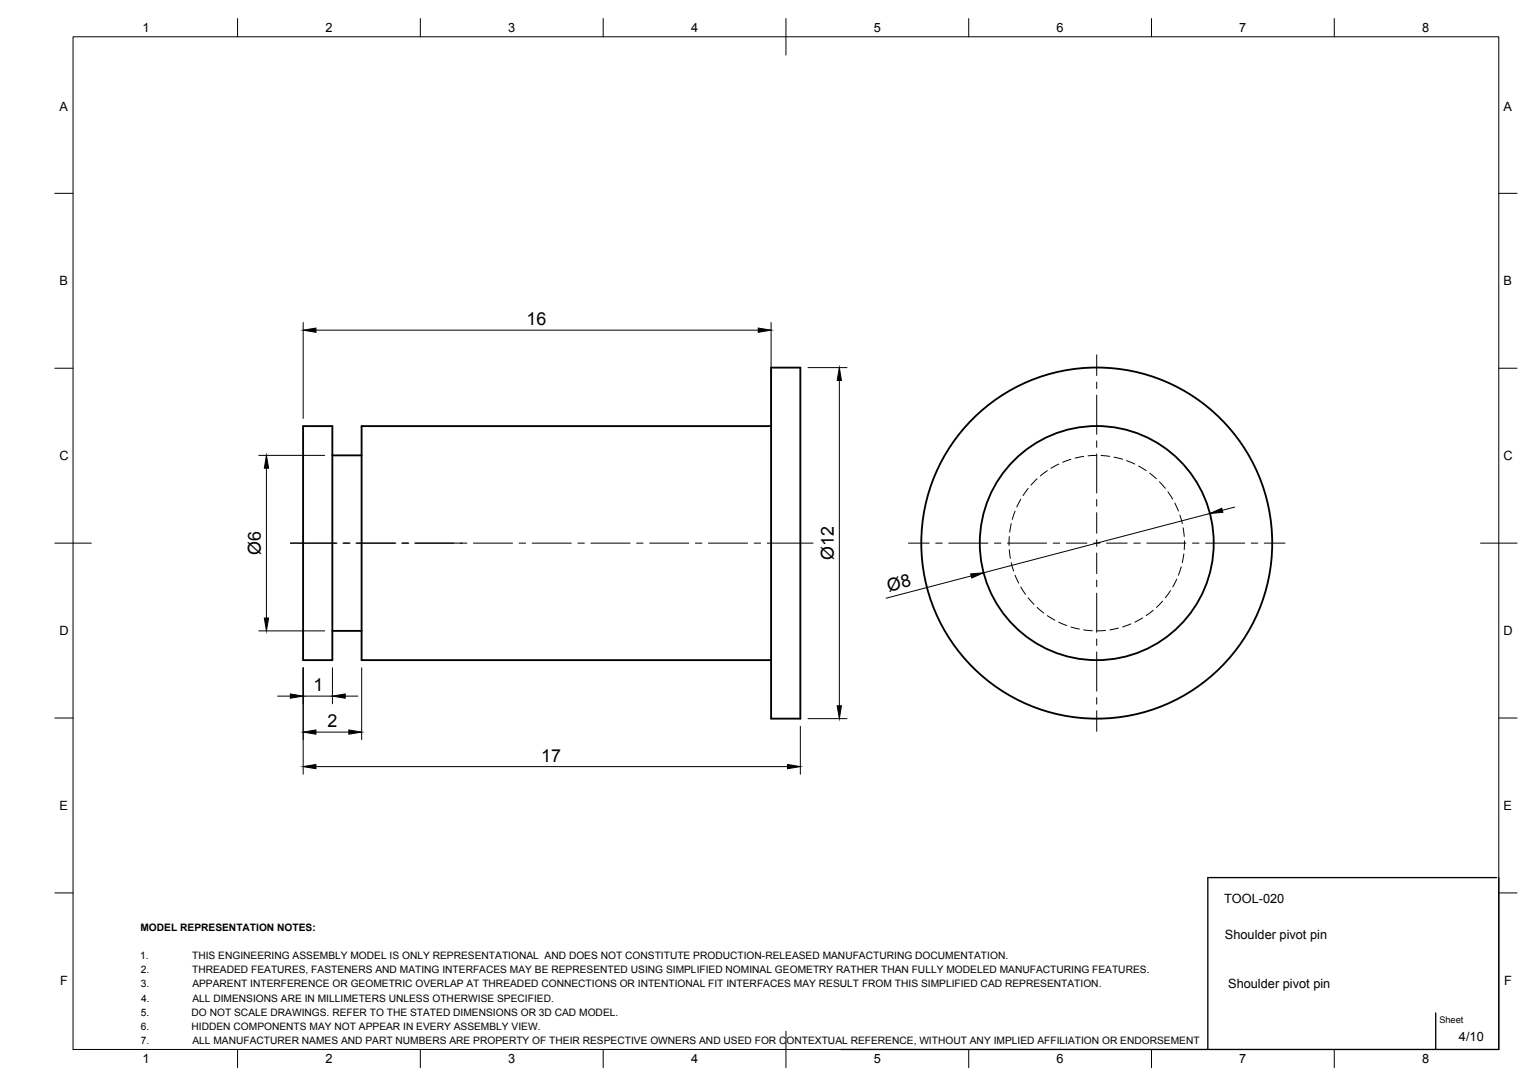
ISO-10303-21;
HEADER;
/* Generated by software containing ST-Developer
 * from STEP Tools, Inc. (www.steptools.com) 
 */

FILE_DESCRIPTION(
/* description */ (''),
/* implementation_level */ '2;1');

FILE_NAME(
/* name */ 'Shoulder pivot pin.step',
/* time_stamp */ '2026-11-10T09:09:39-08:00',
/* author */ (''),
/* organization */ (''),
/* preprocessor_version */ 'ST-DEVELOPER v20.2',
/* originating_system */ 'Autodesk Translation Framework v15.17.0.0',
/* authorisation */ '');

FILE_SCHEMA (('AUTOMOTIVE_DESIGN { 1 0 10303 214 3 1 1 }'));
ENDSEC;

DATA;
#10=MECHANICAL_DESIGN_GEOMETRIC_PRESENTATION_REPRESENTATION('',(#556),#18353);
#538=SHAPE_REPRESENTATION_RELATIONSHIP('SRR','None',#18398,#547);
#547=ADVANCED_BREP_SHAPE_REPRESENTATION('',(#565),#18344);
#556=STYLED_ITEM('',(#18457),#565);
#565=MANIFOLD_SOLID_BREP('Body1',#6487);
#583=FACE_BOUND('',#1197,.T.);
#584=FACE_BOUND('',#1199,.T.);
#585=FACE_BOUND('',#1202,.T.);
#659=PLANE('',#6660);
#660=PLANE('',#6662);
#661=PLANE('',#6666);
#662=PLANE('',#6671);
#663=PLANE('',#6673);
#814=FACE_OUTER_BOUND('',#1195,.T.);
#815=FACE_OUTER_BOUND('',#1196,.T.);
#816=FACE_OUTER_BOUND('',#1198,.T.);
#817=FACE_OUTER_BOUND('',#1200,.T.);
#818=FACE_OUTER_BOUND('',#1201,.T.);
#819=FACE_OUTER_BOUND('',#1203,.T.);
#820=FACE_OUTER_BOUND('',#1204,.T.);
#821=FACE_OUTER_BOUND('',#1205,.T.);
#822=FACE_OUTER_BOUND('',#1206,.T.);
#1195=EDGE_LOOP('',(#4282,#4283,#4284,#4285));
#1196=EDGE_LOOP('',(#4286));
#1197=EDGE_LOOP('',(#4287));
#1198=EDGE_LOOP('',(#4288));
#1199=EDGE_LOOP('',(#4289));
#1200=EDGE_LOOP('',(#4290,#4291,#4292,#4293));
#1201=EDGE_LOOP('',(#4294));
#1202=EDGE_LOOP('',(#4295));
#1203=EDGE_LOOP('',(#4296,#4297,#4298,#4299));
#1204=EDGE_LOOP('',(#4300));
#1205=EDGE_LOOP('',(#4301,#4302,#4303,#4304));
#1206=EDGE_LOOP('',(#4305));
#1651=LINE('',#8643,#2055);
#1652=LINE('',#8654,#2056);
#1653=LINE('',#8662,#2057);
#1654=LINE('',#8666,#2058);
#2055=VECTOR('',#7270,0.3);
#2056=VECTOR('',#7285,0.4);
#2057=VECTOR('',#7294,0.6);
#2058=VECTOR('',#7301,0.4);
#2426=CIRCLE('',#6658,0.3);
#2427=CIRCLE('',#6659,0.3);
#2428=CIRCLE('',#6661,0.4);
#2429=CIRCLE('',#6663,0.4);
#2430=CIRCLE('',#6665,0.4);
#2431=CIRCLE('',#6667,0.6);
#2432=CIRCLE('',#6668,0.4);
#2433=CIRCLE('',#6670,0.6);
#2623=VERTEX_POINT('',#8640);
#2624=VERTEX_POINT('',#8642);
#2625=VERTEX_POINT('',#8646);
#2626=VERTEX_POINT('',#8649);
#2627=VERTEX_POINT('',#8652);
#2628=VERTEX_POINT('',#8656);
#2629=VERTEX_POINT('',#8658);
#2630=VERTEX_POINT('',#8661);
#3258=EDGE_CURVE('',#2623,#2623,#2426,.T.);
#3259=EDGE_CURVE('',#2623,#2624,#1651,.T.);
#3260=EDGE_CURVE('',#2624,#2624,#2427,.T.);
#3261=EDGE_CURVE('',#2625,#2625,#2428,.T.);
#3262=EDGE_CURVE('',#2626,#2626,#2429,.T.);
#3263=EDGE_CURVE('',#2627,#2627,#2430,.T.);
#3264=EDGE_CURVE('',#2627,#2626,#1652,.T.);
#3265=EDGE_CURVE('',#2628,#2628,#2431,.T.);
#3266=EDGE_CURVE('',#2629,#2629,#2432,.T.);
#3267=EDGE_CURVE('',#2628,#2630,#1653,.T.);
#3268=EDGE_CURVE('',#2630,#2630,#2433,.T.);
#3269=EDGE_CURVE('',#2625,#2629,#1654,.T.);
#4282=ORIENTED_EDGE('',*,*,#3258,.T.);
#4283=ORIENTED_EDGE('',*,*,#3259,.T.);
#4284=ORIENTED_EDGE('',*,*,#3260,.F.);
#4285=ORIENTED_EDGE('',*,*,#3259,.F.);
#4286=ORIENTED_EDGE('',*,*,#3261,.F.);
#4287=ORIENTED_EDGE('',*,*,#3258,.F.);
#4288=ORIENTED_EDGE('',*,*,#3262,.F.);
#4289=ORIENTED_EDGE('',*,*,#3260,.T.);
#4290=ORIENTED_EDGE('',*,*,#3263,.F.);
#4291=ORIENTED_EDGE('',*,*,#3264,.T.);
#4292=ORIENTED_EDGE('',*,*,#3262,.T.);
#4293=ORIENTED_EDGE('',*,*,#3264,.F.);
#4294=ORIENTED_EDGE('',*,*,#3265,.T.);
#4295=ORIENTED_EDGE('',*,*,#3266,.F.);
#4296=ORIENTED_EDGE('',*,*,#3265,.F.);
#4297=ORIENTED_EDGE('',*,*,#3267,.T.);
#4298=ORIENTED_EDGE('',*,*,#3268,.T.);
#4299=ORIENTED_EDGE('',*,*,#3267,.F.);
#4300=ORIENTED_EDGE('',*,*,#3268,.F.);
#4301=ORIENTED_EDGE('',*,*,#3261,.T.);
#4302=ORIENTED_EDGE('',*,*,#3269,.T.);
#4303=ORIENTED_EDGE('',*,*,#3266,.T.);
#4304=ORIENTED_EDGE('',*,*,#3269,.F.);
#4305=ORIENTED_EDGE('',*,*,#3263,.T.);
#5992=CYLINDRICAL_SURFACE('',#6657,0.3);
#5993=CYLINDRICAL_SURFACE('',#6664,0.4);
#5994=CYLINDRICAL_SURFACE('',#6669,0.6);
#5995=CYLINDRICAL_SURFACE('',#6672,0.4);
#6145=ADVANCED_FACE('',(#814),#5992,.T.);
#6146=ADVANCED_FACE('',(#815,#583),#659,.F.);
#6147=ADVANCED_FACE('',(#816,#584),#660,.F.);
#6148=ADVANCED_FACE('',(#817),#5993,.T.);
#6149=ADVANCED_FACE('',(#818,#585),#661,.T.);
#6150=ADVANCED_FACE('',(#819),#5994,.T.);
#6151=ADVANCED_FACE('',(#820),#662,.F.);
#6152=ADVANCED_FACE('',(#821),#5995,.T.);
#6153=ADVANCED_FACE('',(#822),#663,.T.);
#6487=CLOSED_SHELL('',(#6145,#6146,#6147,#6148,#6149,#6150,#6151,#6152,
#6153));
#6656=AXIS2_PLACEMENT_3D('',#8638,#7264,#7265);
#6657=AXIS2_PLACEMENT_3D('',#8639,#7266,#7267);
#6658=AXIS2_PLACEMENT_3D('',#8641,#7268,#7269);
#6659=AXIS2_PLACEMENT_3D('',#8644,#7271,#7272);
#6660=AXIS2_PLACEMENT_3D('',#8645,#7273,#7274);
#6661=AXIS2_PLACEMENT_3D('',#8647,#7275,#7276);
#6662=AXIS2_PLACEMENT_3D('',#8648,#7277,#7278);
#6663=AXIS2_PLACEMENT_3D('',#8650,#7279,#7280);
#6664=AXIS2_PLACEMENT_3D('',#8651,#7281,#7282);
#6665=AXIS2_PLACEMENT_3D('',#8653,#7283,#7284);
#6666=AXIS2_PLACEMENT_3D('',#8655,#7286,#7287);
#6667=AXIS2_PLACEMENT_3D('',#8657,#7288,#7289);
#6668=AXIS2_PLACEMENT_3D('',#8659,#7290,#7291);
#6669=AXIS2_PLACEMENT_3D('',#8660,#7292,#7293);
#6670=AXIS2_PLACEMENT_3D('',#8663,#7295,#7296);
#6671=AXIS2_PLACEMENT_3D('',#8664,#7297,#7298);
#6672=AXIS2_PLACEMENT_3D('',#8665,#7299,#7300);
#6673=AXIS2_PLACEMENT_3D('',#8667,#7302,#7303);
#7264=DIRECTION('axis',(0.,0.,1.));
#7265=DIRECTION('refdir',(1.,0.,0.));
#7266=DIRECTION('center_axis',(0.,0.,1.));
#7267=DIRECTION('ref_axis',(1.,0.,0.));
#7268=DIRECTION('center_axis',(0.,0.,1.));
#7269=DIRECTION('ref_axis',(1.,0.,0.));
#7270=DIRECTION('',(0.,0.,1.));
#7271=DIRECTION('center_axis',(0.,0.,1.));
#7272=DIRECTION('ref_axis',(1.,0.,0.));
#7273=DIRECTION('center_axis',(0.,0.,-1.));
#7274=DIRECTION('ref_axis',(-1.,0.,0.));
#7275=DIRECTION('center_axis',(0.,0.,-1.));
#7276=DIRECTION('ref_axis',(1.,0.,0.));
#7277=DIRECTION('center_axis',(0.,0.,1.));
#7278=DIRECTION('ref_axis',(1.,0.,0.));
#7279=DIRECTION('center_axis',(0.,0.,1.));
#7280=DIRECTION('ref_axis',(1.,0.,0.));
#7281=DIRECTION('center_axis',(0.,0.,1.));
#7282=DIRECTION('ref_axis',(1.,0.,0.));
#7283=DIRECTION('center_axis',(0.,0.,1.));
#7284=DIRECTION('ref_axis',(1.,0.,0.));
#7285=DIRECTION('',(0.,0.,-1.));
#7286=DIRECTION('center_axis',(0.,0.,1.));
#7287=DIRECTION('ref_axis',(1.,0.,0.));
#7288=DIRECTION('center_axis',(0.,0.,1.));
#7289=DIRECTION('ref_axis',(1.,0.,0.));
#7290=DIRECTION('center_axis',(0.,0.,1.));
#7291=DIRECTION('ref_axis',(1.,0.,0.));
#7292=DIRECTION('center_axis',(0.,0.,1.));
#7293=DIRECTION('ref_axis',(1.,0.,0.));
#7294=DIRECTION('',(0.,0.,-1.));
#7295=DIRECTION('center_axis',(0.,0.,1.));
#7296=DIRECTION('ref_axis',(1.,0.,0.));
#7297=DIRECTION('center_axis',(0.,0.,1.));
#7298=DIRECTION('ref_axis',(1.,0.,0.));
#7299=DIRECTION('center_axis',(0.,0.,1.));
#7300=DIRECTION('ref_axis',(1.,0.,0.));
#7301=DIRECTION('',(0.,0.,-1.));
#7302=DIRECTION('center_axis',(0.,0.,1.));
#7303=DIRECTION('ref_axis',(1.,0.,0.));
#8638=CARTESIAN_POINT('',(0.,0.,0.));
#8639=CARTESIAN_POINT('Origin',(0.,0.,0.75));
#8640=CARTESIAN_POINT('',(-0.3,-3.67394039744206E-17,0.7));
#8641=CARTESIAN_POINT('Origin',(0.,0.,0.7));
#8642=CARTESIAN_POINT('',(-0.3,-3.67394039744206E-17,0.8));
#8643=CARTESIAN_POINT('',(-0.3,-3.67394039744206E-17,0.75));
#8644=CARTESIAN_POINT('Origin',(0.,0.,0.8));
#8645=CARTESIAN_POINT('Origin',(0.7,0.,0.7));
#8646=CARTESIAN_POINT('',(-0.4,4.89858719658941E-17,0.7));
#8647=CARTESIAN_POINT('Origin',(0.,0.,0.7));
#8648=CARTESIAN_POINT('Origin',(0.3,0.,0.8));
#8649=CARTESIAN_POINT('',(-0.4,-4.89858719658941E-17,0.8));
#8650=CARTESIAN_POINT('Origin',(0.,0.,0.8));
#8651=CARTESIAN_POINT('Origin',(0.,0.,-0.7));
#8652=CARTESIAN_POINT('',(-0.4,-4.89858719658941E-17,0.9));
#8653=CARTESIAN_POINT('Origin',(0.,0.,0.9));
#8654=CARTESIAN_POINT('',(-0.4,-4.89858719658941E-17,-0.7));
#8655=CARTESIAN_POINT('Origin',(0.,0.,-0.7));
#8656=CARTESIAN_POINT('',(-0.6,-7.34788079488412E-17,-0.7));
#8657=CARTESIAN_POINT('Origin',(0.,0.,-0.7));
#8658=CARTESIAN_POINT('',(-0.4,-4.89858719658941E-17,-0.7));
#8659=CARTESIAN_POINT('Origin',(0.,0.,-0.7));
#8660=CARTESIAN_POINT('Origin',(0.,0.,-0.8));
#8661=CARTESIAN_POINT('',(-0.6,-7.34788079488412E-17,-0.8));
#8662=CARTESIAN_POINT('',(-0.6,-7.34788079488412E-17,-0.8));
#8663=CARTESIAN_POINT('Origin',(0.,0.,-0.8));
#8664=CARTESIAN_POINT('Origin',(0.,0.,-0.8));
#8665=CARTESIAN_POINT('Origin',(0.,0.,-0.7));
#8666=CARTESIAN_POINT('',(-0.4,-4.89858719658941E-17,-0.7));
#8667=CARTESIAN_POINT('Origin',(0.,0.,0.9));
#18332=UNCERTAINTY_MEASURE_WITH_UNIT(LENGTH_MEASURE(0.001),#18354,
'DISTANCE_ACCURACY_VALUE',
'Maximum model space distance between geometric entities at asserted c
onnectivities');
#18341=UNCERTAINTY_MEASURE_WITH_UNIT(LENGTH_MEASURE(0.001),#18354,
'DISTANCE_ACCURACY_VALUE',
'Maximum model space distance between geometric entities at asserted c
onnectivities');
#18344=(
GEOMETRIC_REPRESENTATION_CONTEXT(3)
GLOBAL_UNCERTAINTY_ASSIGNED_CONTEXT((#18332))
GLOBAL_UNIT_ASSIGNED_CONTEXT((#18354,#18356,#18357))
REPRESENTATION_CONTEXT('','3D')
);
#18353=(
GEOMETRIC_REPRESENTATION_CONTEXT(3)
GLOBAL_UNCERTAINTY_ASSIGNED_CONTEXT((#18341))
GLOBAL_UNIT_ASSIGNED_CONTEXT((#18354,#18356,#18357))
REPRESENTATION_CONTEXT('','3D')
);
#18354=(
LENGTH_UNIT()
NAMED_UNIT(*)
SI_UNIT(.CENTI.,.METRE.)
);
#18356=(
NAMED_UNIT(*)
PLANE_ANGLE_UNIT()
SI_UNIT($,.RADIAN.)
);
#18357=(
NAMED_UNIT(*)
SI_UNIT($,.STERADIAN.)
SOLID_ANGLE_UNIT()
);
#18360=SHAPE_DEFINITION_REPRESENTATION(#18371,#18398);
#18371=PRODUCT_DEFINITION_SHAPE('',$,#18410);
#18398=SHAPE_REPRESENTATION('',(#6656),#18344);
#18407=PRODUCT_DEFINITION_CONTEXT('part definition',#18442,'design');
#18410=PRODUCT_DEFINITION('Shoulder pivot pin','Shoulder pivot pin',#18421,
#18407);
#18421=PRODUCT_DEFINITION_FORMATION('',$,#18446);
#18442=APPLICATION_CONTEXT(
'Core Data for Automotive Mechanical Design Process');
#18443=PRODUCT_CONTEXT('part definition',#18442,'mechanical');
#18446=PRODUCT('Shoulder pivot pin','Shoulder pivot pin',$,(#18443));
#18457=PRESENTATION_STYLE_ASSIGNMENT((#18465));
#18465=SURFACE_STYLE_USAGE(.BOTH.,#18473);
#18473=SURFACE_SIDE_STYLE('',(#18481));
#18481=SURFACE_STYLE_FILL_AREA(#18489);
#18489=FILL_AREA_STYLE('Pivot dark gray',(#18497));
#18497=FILL_AREA_STYLE_COLOUR('Pivot dark gray',#18505);
#18505=COLOUR_RGB('Pivot dark gray',0.27843137254902,0.309803921568627,
0.352941176470588);
ENDSEC;
END-ISO-10303-21;
